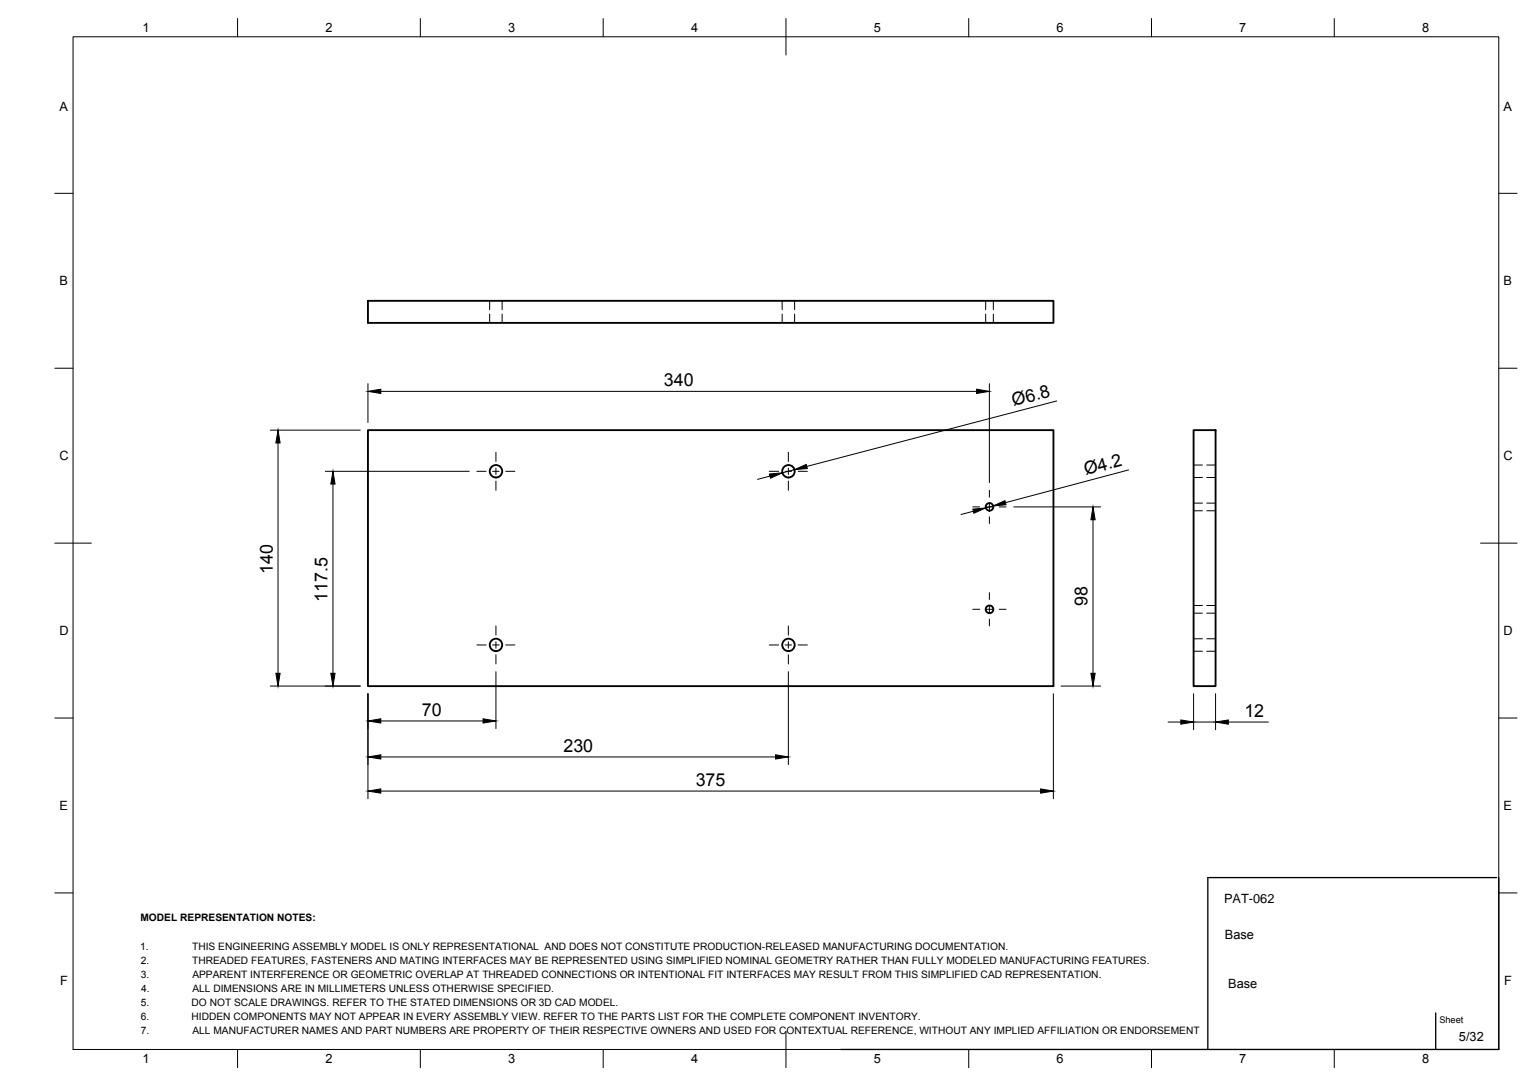
ISO-10303-21;
HEADER;
/* Generated by software containing ST-Developer
 * from STEP Tools, Inc. (www.steptools.com) 
 */

FILE_DESCRIPTION(
/* description */ ('Jaw-coupled motor to shaft test stand'),
/* implementation_level */ '2;1');

FILE_NAME(
/* name */ 'Base.step',
/* time_stamp */ '2026-10-27T10:46:06-07:00',
/* author */ (''),
/* organization */ (''),
/* preprocessor_version */ 'ST-DEVELOPER v20.2',
/* originating_system */ 'Autodesk Translation Framework v15.17.0.0',
/* authorisation */ '');

FILE_SCHEMA (('AUTOMOTIVE_DESIGN { 1 0 10303 214 3 1 1 }'));
ENDSEC;

DATA;
#10=MECHANICAL_DESIGN_GEOMETRIC_PRESENTATION_REPRESENTATION('',(#340),#19361);
#276=SHAPE_REPRESENTATION_RELATIONSHIP('SRR','None',#19490,#308);
#308=ADVANCED_BREP_SHAPE_REPRESENTATION('',(#373),#19326);
#340=STYLED_ITEM('',(#19725),#373);
#373=MANIFOLD_SOLID_BREP('Body1',#10984);
#403=FACE_BOUND('',#1653,.T.);
#404=FACE_BOUND('',#1654,.T.);
#405=FACE_BOUND('',#1655,.T.);
#406=FACE_BOUND('',#1656,.T.);
#407=FACE_BOUND('',#1657,.T.);
#408=FACE_BOUND('',#1658,.T.);
#409=FACE_BOUND('',#1660,.T.);
#410=FACE_BOUND('',#1661,.T.);
#411=FACE_BOUND('',#1662,.T.);
#412=FACE_BOUND('',#1663,.T.);
#413=FACE_BOUND('',#1664,.T.);
#414=FACE_BOUND('',#1665,.T.);
#516=PLANE('',#11394);
#517=PLANE('',#11395);
#518=PLANE('',#11396);
#519=PLANE('',#11397);
#520=PLANE('',#11398);
#521=PLANE('',#11399);
#1022=FACE_OUTER_BOUND('',#1642,.T.);
#1023=FACE_OUTER_BOUND('',#1643,.T.);
#1024=FACE_OUTER_BOUND('',#1644,.T.);
#1025=FACE_OUTER_BOUND('',#1645,.T.);
#1026=FACE_OUTER_BOUND('',#1646,.T.);
#1027=FACE_OUTER_BOUND('',#1647,.T.);
#1028=FACE_OUTER_BOUND('',#1648,.T.);
#1029=FACE_OUTER_BOUND('',#1649,.T.);
#1030=FACE_OUTER_BOUND('',#1650,.T.);
#1031=FACE_OUTER_BOUND('',#1651,.T.);
#1032=FACE_OUTER_BOUND('',#1652,.T.);
#1033=FACE_OUTER_BOUND('',#1659,.T.);
#1642=EDGE_LOOP('',(#7346,#7347,#7348,#7349));
#1643=EDGE_LOOP('',(#7350,#7351,#7352,#7353));
#1644=EDGE_LOOP('',(#7354,#7355,#7356,#7357));
#1645=EDGE_LOOP('',(#7358,#7359,#7360,#7361));
#1646=EDGE_LOOP('',(#7362,#7363,#7364,#7365));
#1647=EDGE_LOOP('',(#7366,#7367,#7368,#7369));
#1648=EDGE_LOOP('',(#7370,#7371,#7372,#7373));
#1649=EDGE_LOOP('',(#7374,#7375,#7376,#7377));
#1650=EDGE_LOOP('',(#7378,#7379,#7380,#7381));
#1651=EDGE_LOOP('',(#7382,#7383,#7384,#7385));
#1652=EDGE_LOOP('',(#7386,#7387,#7388,#7389));
#1653=EDGE_LOOP('',(#7390));
#1654=EDGE_LOOP('',(#7391));
#1655=EDGE_LOOP('',(#7392));
#1656=EDGE_LOOP('',(#7393));
#1657=EDGE_LOOP('',(#7394));
#1658=EDGE_LOOP('',(#7395));
#1659=EDGE_LOOP('',(#7396,#7397,#7398,#7399));
#1660=EDGE_LOOP('',(#7400));
#1661=EDGE_LOOP('',(#7401));
#1662=EDGE_LOOP('',(#7402));
#1663=EDGE_LOOP('',(#7403));
#1664=EDGE_LOOP('',(#7404));
#1665=EDGE_LOOP('',(#7405));
#2375=LINE('',#15434,#3528);
#2376=LINE('',#15440,#3529);
#2377=LINE('',#15446,#3530);
#2378=LINE('',#15452,#3531);
#2379=LINE('',#15458,#3532);
#2380=LINE('',#15464,#3533);
#2381=LINE('',#15469,#3534);
#2382=LINE('',#15471,#3535);
#2383=LINE('',#15473,#3536);
#2384=LINE('',#15474,#3537);
#2385=LINE('',#15477,#3538);
#2386=LINE('',#15479,#3539);
#2387=LINE('',#15480,#3540);
#2388=LINE('',#15483,#3541);
#2389=LINE('',#15485,#3542);
#2390=LINE('',#15486,#3543);
#2391=LINE('',#15488,#3544);
#2392=LINE('',#15489,#3545);
#3528=VECTOR('',#12350,0.21);
#3529=VECTOR('',#12357,0.21);
#3530=VECTOR('',#12364,0.34);
#3531=VECTOR('',#12371,0.34);
#3532=VECTOR('',#12378,0.34);
#3533=VECTOR('',#12385,0.34);
#3534=VECTOR('',#12390,1.);
#3535=VECTOR('',#12391,1.);
#3536=VECTOR('',#12392,1.);
#3537=VECTOR('',#12393,1.);
#3538=VECTOR('',#12396,1.);
#3539=VECTOR('',#12397,1.);
#3540=VECTOR('',#12398,1.);
#3541=VECTOR('',#12401,1.);
#3542=VECTOR('',#12402,1.);
#3543=VECTOR('',#12403,1.);
#3544=VECTOR('',#12406,1.);
#3545=VECTOR('',#12407,1.);
#4681=CIRCLE('',#11377,0.21);
#4682=CIRCLE('',#11378,0.21);
#4683=CIRCLE('',#11380,0.21);
#4684=CIRCLE('',#11381,0.21);
#4685=CIRCLE('',#11383,0.34);
#4686=CIRCLE('',#11384,0.34);
#4687=CIRCLE('',#11386,0.34);
#4688=CIRCLE('',#11387,0.34);
#4689=CIRCLE('',#11389,0.34);
#4690=CIRCLE('',#11390,0.34);
#4691=CIRCLE('',#11392,0.34);
#4692=CIRCLE('',#11393,0.34);
#4943=VERTEX_POINT('',#15431);
#4944=VERTEX_POINT('',#15433);
#4945=VERTEX_POINT('',#15437);
#4946=VERTEX_POINT('',#15439);
#4947=VERTEX_POINT('',#15443);
#4948=VERTEX_POINT('',#15445);
#4949=VERTEX_POINT('',#15449);
#4950=VERTEX_POINT('',#15451);
#4951=VERTEX_POINT('',#15455);
#4952=VERTEX_POINT('',#15457);
#4953=VERTEX_POINT('',#15461);
#4954=VERTEX_POINT('',#15463);
#4955=VERTEX_POINT('',#15467);
#4956=VERTEX_POINT('',#15468);
#4957=VERTEX_POINT('',#15470);
#4958=VERTEX_POINT('',#15472);
#4959=VERTEX_POINT('',#15476);
#4960=VERTEX_POINT('',#15478);
#4961=VERTEX_POINT('',#15482);
#4962=VERTEX_POINT('',#15484);
#5884=EDGE_CURVE('',#4943,#4943,#4681,.T.);
#5885=EDGE_CURVE('',#4943,#4944,#2375,.T.);
#5886=EDGE_CURVE('',#4944,#4944,#4682,.T.);
#5887=EDGE_CURVE('',#4945,#4945,#4683,.T.);
#5888=EDGE_CURVE('',#4945,#4946,#2376,.T.);
#5889=EDGE_CURVE('',#4946,#4946,#4684,.T.);
#5890=EDGE_CURVE('',#4947,#4947,#4685,.T.);
#5891=EDGE_CURVE('',#4947,#4948,#2377,.T.);
#5892=EDGE_CURVE('',#4948,#4948,#4686,.T.);
#5893=EDGE_CURVE('',#4949,#4949,#4687,.T.);
#5894=EDGE_CURVE('',#4949,#4950,#2378,.T.);
#5895=EDGE_CURVE('',#4950,#4950,#4688,.T.);
#5896=EDGE_CURVE('',#4951,#4951,#4689,.T.);
#5897=EDGE_CURVE('',#4951,#4952,#2379,.T.);
#5898=EDGE_CURVE('',#4952,#4952,#4690,.T.);
#5899=EDGE_CURVE('',#4953,#4953,#4691,.T.);
#5900=EDGE_CURVE('',#4953,#4954,#2380,.T.);
#5901=EDGE_CURVE('',#4954,#4954,#4692,.T.);
#5902=EDGE_CURVE('',#4955,#4956,#2381,.T.);
#5903=EDGE_CURVE('',#4956,#4957,#2382,.T.);
#5904=EDGE_CURVE('',#4958,#4957,#2383,.T.);
#5905=EDGE_CURVE('',#4955,#4958,#2384,.T.);
#5906=EDGE_CURVE('',#4959,#4955,#2385,.T.);
#5907=EDGE_CURVE('',#4960,#4958,#2386,.T.);
#5908=EDGE_CURVE('',#4959,#4960,#2387,.T.);
#5909=EDGE_CURVE('',#4961,#4959,#2388,.T.);
#5910=EDGE_CURVE('',#4962,#4960,#2389,.T.);
#5911=EDGE_CURVE('',#4961,#4962,#2390,.T.);
#5912=EDGE_CURVE('',#4956,#4961,#2391,.T.);
#5913=EDGE_CURVE('',#4957,#4962,#2392,.T.);
#7346=ORIENTED_EDGE('',*,*,#5884,.F.);
#7347=ORIENTED_EDGE('',*,*,#5885,.T.);
#7348=ORIENTED_EDGE('',*,*,#5886,.F.);
#7349=ORIENTED_EDGE('',*,*,#5885,.F.);
#7350=ORIENTED_EDGE('',*,*,#5887,.F.);
#7351=ORIENTED_EDGE('',*,*,#5888,.T.);
#7352=ORIENTED_EDGE('',*,*,#5889,.F.);
#7353=ORIENTED_EDGE('',*,*,#5888,.F.);
#7354=ORIENTED_EDGE('',*,*,#5890,.F.);
#7355=ORIENTED_EDGE('',*,*,#5891,.T.);
#7356=ORIENTED_EDGE('',*,*,#5892,.F.);
#7357=ORIENTED_EDGE('',*,*,#5891,.F.);
#7358=ORIENTED_EDGE('',*,*,#5893,.F.);
#7359=ORIENTED_EDGE('',*,*,#5894,.T.);
#7360=ORIENTED_EDGE('',*,*,#5895,.F.);
#7361=ORIENTED_EDGE('',*,*,#5894,.F.);
#7362=ORIENTED_EDGE('',*,*,#5896,.F.);
#7363=ORIENTED_EDGE('',*,*,#5897,.T.);
#7364=ORIENTED_EDGE('',*,*,#5898,.F.);
#7365=ORIENTED_EDGE('',*,*,#5897,.F.);
#7366=ORIENTED_EDGE('',*,*,#5899,.F.);
#7367=ORIENTED_EDGE('',*,*,#5900,.T.);
#7368=ORIENTED_EDGE('',*,*,#5901,.F.);
#7369=ORIENTED_EDGE('',*,*,#5900,.F.);
#7370=ORIENTED_EDGE('',*,*,#5902,.T.);
#7371=ORIENTED_EDGE('',*,*,#5903,.T.);
#7372=ORIENTED_EDGE('',*,*,#5904,.F.);
#7373=ORIENTED_EDGE('',*,*,#5905,.F.);
#7374=ORIENTED_EDGE('',*,*,#5906,.T.);
#7375=ORIENTED_EDGE('',*,*,#5905,.T.);
#7376=ORIENTED_EDGE('',*,*,#5907,.F.);
#7377=ORIENTED_EDGE('',*,*,#5908,.F.);
#7378=ORIENTED_EDGE('',*,*,#5909,.T.);
#7379=ORIENTED_EDGE('',*,*,#5908,.T.);
#7380=ORIENTED_EDGE('',*,*,#5910,.F.);
#7381=ORIENTED_EDGE('',*,*,#5911,.F.);
#7382=ORIENTED_EDGE('',*,*,#5912,.T.);
#7383=ORIENTED_EDGE('',*,*,#5911,.T.);
#7384=ORIENTED_EDGE('',*,*,#5913,.F.);
#7385=ORIENTED_EDGE('',*,*,#5903,.F.);
#7386=ORIENTED_EDGE('',*,*,#5913,.T.);
#7387=ORIENTED_EDGE('',*,*,#5910,.T.);
#7388=ORIENTED_EDGE('',*,*,#5907,.T.);
#7389=ORIENTED_EDGE('',*,*,#5904,.T.);
#7390=ORIENTED_EDGE('',*,*,#5886,.T.);
#7391=ORIENTED_EDGE('',*,*,#5889,.T.);
#7392=ORIENTED_EDGE('',*,*,#5892,.T.);
#7393=ORIENTED_EDGE('',*,*,#5895,.T.);
#7394=ORIENTED_EDGE('',*,*,#5898,.T.);
#7395=ORIENTED_EDGE('',*,*,#5901,.T.);
#7396=ORIENTED_EDGE('',*,*,#5912,.F.);
#7397=ORIENTED_EDGE('',*,*,#5902,.F.);
#7398=ORIENTED_EDGE('',*,*,#5906,.F.);
#7399=ORIENTED_EDGE('',*,*,#5909,.F.);
#7400=ORIENTED_EDGE('',*,*,#5884,.T.);
#7401=ORIENTED_EDGE('',*,*,#5887,.T.);
#7402=ORIENTED_EDGE('',*,*,#5890,.T.);
#7403=ORIENTED_EDGE('',*,*,#5893,.T.);
#7404=ORIENTED_EDGE('',*,*,#5896,.T.);
#7405=ORIENTED_EDGE('',*,*,#5899,.T.);
#10270=CYLINDRICAL_SURFACE('',#11376,0.21);
#10271=CYLINDRICAL_SURFACE('',#11379,0.21);
#10272=CYLINDRICAL_SURFACE('',#11382,0.34);
#10273=CYLINDRICAL_SURFACE('',#11385,0.34);
#10274=CYLINDRICAL_SURFACE('',#11388,0.34);
#10275=CYLINDRICAL_SURFACE('',#11391,0.34);
#10364=ADVANCED_FACE('',(#1022),#10270,.F.);
#10365=ADVANCED_FACE('',(#1023),#10271,.F.);
#10366=ADVANCED_FACE('',(#1024),#10272,.F.);
#10367=ADVANCED_FACE('',(#1025),#10273,.F.);
#10368=ADVANCED_FACE('',(#1026),#10274,.F.);
#10369=ADVANCED_FACE('',(#1027),#10275,.F.);
#10370=ADVANCED_FACE('',(#1028),#516,.T.);
#10371=ADVANCED_FACE('',(#1029),#517,.T.);
#10372=ADVANCED_FACE('',(#1030),#518,.T.);
#10373=ADVANCED_FACE('',(#1031),#519,.T.);
#10374=ADVANCED_FACE('',(#1032,#403,#404,#405,#406,#407,#408),#520,.T.);
#10375=ADVANCED_FACE('',(#1033,#409,#410,#411,#412,#413,#414),#521,.F.);
#10984=CLOSED_SHELL('',(#10364,#10365,#10366,#10367,#10368,#10369,#10370,
#10371,#10372,#10373,#10374,#10375));
#11375=AXIS2_PLACEMENT_3D('',#15429,#12344,#12345);
#11376=AXIS2_PLACEMENT_3D('',#15430,#12346,#12347);
#11377=AXIS2_PLACEMENT_3D('',#15432,#12348,#12349);
#11378=AXIS2_PLACEMENT_3D('',#15435,#12351,#12352);
#11379=AXIS2_PLACEMENT_3D('',#15436,#12353,#12354);
#11380=AXIS2_PLACEMENT_3D('',#15438,#12355,#12356);
#11381=AXIS2_PLACEMENT_3D('',#15441,#12358,#12359);
#11382=AXIS2_PLACEMENT_3D('',#15442,#12360,#12361);
#11383=AXIS2_PLACEMENT_3D('',#15444,#12362,#12363);
#11384=AXIS2_PLACEMENT_3D('',#15447,#12365,#12366);
#11385=AXIS2_PLACEMENT_3D('',#15448,#12367,#12368);
#11386=AXIS2_PLACEMENT_3D('',#15450,#12369,#12370);
#11387=AXIS2_PLACEMENT_3D('',#15453,#12372,#12373);
#11388=AXIS2_PLACEMENT_3D('',#15454,#12374,#12375);
#11389=AXIS2_PLACEMENT_3D('',#15456,#12376,#12377);
#11390=AXIS2_PLACEMENT_3D('',#15459,#12379,#12380);
#11391=AXIS2_PLACEMENT_3D('',#15460,#12381,#12382);
#11392=AXIS2_PLACEMENT_3D('',#15462,#12383,#12384);
#11393=AXIS2_PLACEMENT_3D('',#15465,#12386,#12387);
#11394=AXIS2_PLACEMENT_3D('',#15466,#12388,#12389);
#11395=AXIS2_PLACEMENT_3D('',#15475,#12394,#12395);
#11396=AXIS2_PLACEMENT_3D('',#15481,#12399,#12400);
#11397=AXIS2_PLACEMENT_3D('',#15487,#12404,#12405);
#11398=AXIS2_PLACEMENT_3D('',#15490,#12408,#12409);
#11399=AXIS2_PLACEMENT_3D('',#15491,#12410,#12411);
#12344=DIRECTION('axis',(0.,0.,1.));
#12345=DIRECTION('refdir',(1.,0.,0.));
#12346=DIRECTION('center_axis',(0.,0.,1.));
#12347=DIRECTION('ref_axis',(1.,0.,0.));
#12348=DIRECTION('center_axis',(0.,0.,1.));
#12349=DIRECTION('ref_axis',(1.,0.,0.));
#12350=DIRECTION('',(0.,0.,1.));
#12351=DIRECTION('center_axis',(0.,0.,-1.));
#12352=DIRECTION('ref_axis',(1.,0.,0.));
#12353=DIRECTION('center_axis',(0.,0.,1.));
#12354=DIRECTION('ref_axis',(1.,0.,0.));
#12355=DIRECTION('center_axis',(0.,0.,1.));
#12356=DIRECTION('ref_axis',(1.,0.,0.));
#12357=DIRECTION('',(0.,0.,1.));
#12358=DIRECTION('center_axis',(0.,0.,-1.));
#12359=DIRECTION('ref_axis',(1.,0.,0.));
#12360=DIRECTION('center_axis',(0.,0.,1.));
#12361=DIRECTION('ref_axis',(1.,0.,0.));
#12362=DIRECTION('center_axis',(0.,0.,1.));
#12363=DIRECTION('ref_axis',(1.,0.,0.));
#12364=DIRECTION('',(0.,0.,1.));
#12365=DIRECTION('center_axis',(0.,0.,-1.));
#12366=DIRECTION('ref_axis',(1.,0.,0.));
#12367=DIRECTION('center_axis',(0.,0.,1.));
#12368=DIRECTION('ref_axis',(1.,0.,0.));
#12369=DIRECTION('center_axis',(0.,0.,1.));
#12370=DIRECTION('ref_axis',(1.,0.,0.));
#12371=DIRECTION('',(0.,0.,1.));
#12372=DIRECTION('center_axis',(0.,0.,-1.));
#12373=DIRECTION('ref_axis',(1.,0.,0.));
#12374=DIRECTION('center_axis',(0.,0.,1.));
#12375=DIRECTION('ref_axis',(1.,0.,0.));
#12376=DIRECTION('center_axis',(0.,0.,1.));
#12377=DIRECTION('ref_axis',(1.,0.,0.));
#12378=DIRECTION('',(0.,0.,1.));
#12379=DIRECTION('center_axis',(0.,0.,-1.));
#12380=DIRECTION('ref_axis',(1.,0.,0.));
#12381=DIRECTION('center_axis',(0.,0.,1.));
#12382=DIRECTION('ref_axis',(1.,0.,0.));
#12383=DIRECTION('center_axis',(0.,0.,1.));
#12384=DIRECTION('ref_axis',(1.,0.,0.));
#12385=DIRECTION('',(0.,0.,1.));
#12386=DIRECTION('center_axis',(0.,0.,-1.));
#12387=DIRECTION('ref_axis',(1.,0.,0.));
#12388=DIRECTION('center_axis',(0.,1.,0.));
#12389=DIRECTION('ref_axis',(-1.,0.,0.));
#12390=DIRECTION('',(-1.,0.,0.));
#12391=DIRECTION('',(0.,0.,1.));
#12392=DIRECTION('',(-1.,0.,0.));
#12393=DIRECTION('',(0.,0.,1.));
#12394=DIRECTION('center_axis',(1.,0.,0.));
#12395=DIRECTION('ref_axis',(0.,1.,0.));
#12396=DIRECTION('',(0.,1.,0.));
#12397=DIRECTION('',(0.,1.,0.));
#12398=DIRECTION('',(0.,0.,1.));
#12399=DIRECTION('center_axis',(0.,-1.,0.));
#12400=DIRECTION('ref_axis',(1.,0.,0.));
#12401=DIRECTION('',(1.,0.,0.));
#12402=DIRECTION('',(1.,0.,0.));
#12403=DIRECTION('',(0.,0.,1.));
#12404=DIRECTION('center_axis',(-1.,0.,0.));
#12405=DIRECTION('ref_axis',(0.,-1.,0.));
#12406=DIRECTION('',(0.,-1.,0.));
#12407=DIRECTION('',(0.,-1.,0.));
#12408=DIRECTION('center_axis',(0.,0.,1.));
#12409=DIRECTION('ref_axis',(1.,0.,0.));
#12410=DIRECTION('center_axis',(0.,0.,1.));
#12411=DIRECTION('ref_axis',(1.,0.,0.));
#15429=CARTESIAN_POINT('',(0.,0.,0.));
#15430=CARTESIAN_POINT('Origin',(-2.8,-9.,-0.1));
#15431=CARTESIAN_POINT('',(-3.01,-9.,0.));
#15432=CARTESIAN_POINT('Origin',(-2.8,-9.,0.));
#15433=CARTESIAN_POINT('',(-3.01,-9.,1.2));
#15434=CARTESIAN_POINT('',(-3.01,-9.,-0.1));
#15435=CARTESIAN_POINT('Origin',(-2.8,-9.,1.2));
#15436=CARTESIAN_POINT('Origin',(2.8,-9.,-0.1));
#15437=CARTESIAN_POINT('',(2.59,-9.,0.));
#15438=CARTESIAN_POINT('Origin',(2.8,-9.,0.));
#15439=CARTESIAN_POINT('',(2.59,-9.,1.2));
#15440=CARTESIAN_POINT('',(2.59,-9.,-0.1));
#15441=CARTESIAN_POINT('Origin',(2.8,-9.,1.2));
#15442=CARTESIAN_POINT('Origin',(4.75,2.,-0.1));
#15443=CARTESIAN_POINT('',(4.41,2.,0.));
#15444=CARTESIAN_POINT('Origin',(4.75,2.,0.));
#15445=CARTESIAN_POINT('',(4.41,2.,1.2));
#15446=CARTESIAN_POINT('',(4.41,2.,-0.1));
#15447=CARTESIAN_POINT('Origin',(4.75,2.,1.2));
#15448=CARTESIAN_POINT('Origin',(-4.75,18.,-0.1));
#15449=CARTESIAN_POINT('',(-5.09,18.,0.));
#15450=CARTESIAN_POINT('Origin',(-4.75,18.,0.));
#15451=CARTESIAN_POINT('',(-5.09,18.,1.2));
#15452=CARTESIAN_POINT('',(-5.09,18.,-0.1));
#15453=CARTESIAN_POINT('Origin',(-4.75,18.,1.2));
#15454=CARTESIAN_POINT('Origin',(-4.75,2.,-0.1));
#15455=CARTESIAN_POINT('',(-5.09,2.,0.));
#15456=CARTESIAN_POINT('Origin',(-4.75,2.,0.));
#15457=CARTESIAN_POINT('',(-5.09,2.,1.2));
#15458=CARTESIAN_POINT('',(-5.09,2.,-0.1));
#15459=CARTESIAN_POINT('Origin',(-4.75,2.,1.2));
#15460=CARTESIAN_POINT('Origin',(4.75,18.,-0.1));
#15461=CARTESIAN_POINT('',(4.41,18.,0.));
#15462=CARTESIAN_POINT('Origin',(4.75,18.,0.));
#15463=CARTESIAN_POINT('',(4.41,18.,1.2));
#15464=CARTESIAN_POINT('',(4.41,18.,-0.1));
#15465=CARTESIAN_POINT('Origin',(4.75,18.,1.2));
#15466=CARTESIAN_POINT('Origin',(7.,25.,0.));
#15467=CARTESIAN_POINT('',(7.,25.,0.));
#15468=CARTESIAN_POINT('',(-7.,25.,0.));
#15469=CARTESIAN_POINT('',(7.,25.,0.));
#15470=CARTESIAN_POINT('',(-7.,25.,1.2));
#15471=CARTESIAN_POINT('',(-7.,25.,0.));
#15472=CARTESIAN_POINT('',(7.,25.,1.2));
#15473=CARTESIAN_POINT('',(7.,25.,1.2));
#15474=CARTESIAN_POINT('',(7.,25.,0.));
#15475=CARTESIAN_POINT('Origin',(7.,-12.5,0.));
#15476=CARTESIAN_POINT('',(7.,-12.5,0.));
#15477=CARTESIAN_POINT('',(7.,-12.5,0.));
#15478=CARTESIAN_POINT('',(7.,-12.5,1.2));
#15479=CARTESIAN_POINT('',(7.,-12.5,1.2));
#15480=CARTESIAN_POINT('',(7.,-12.5,0.));
#15481=CARTESIAN_POINT('Origin',(-7.,-12.5,0.));
#15482=CARTESIAN_POINT('',(-7.,-12.5,0.));
#15483=CARTESIAN_POINT('',(-7.,-12.5,0.));
#15484=CARTESIAN_POINT('',(-7.,-12.5,1.2));
#15485=CARTESIAN_POINT('',(-7.,-12.5,1.2));
#15486=CARTESIAN_POINT('',(-7.,-12.5,0.));
#15487=CARTESIAN_POINT('Origin',(-7.,25.,0.));
#15488=CARTESIAN_POINT('',(-7.,25.,0.));
#15489=CARTESIAN_POINT('',(-7.,25.,1.2));
#15490=CARTESIAN_POINT('Origin',(0.,6.25,1.2));
#15491=CARTESIAN_POINT('Origin',(0.,6.25,0.));
#19288=UNCERTAINTY_MEASURE_WITH_UNIT(LENGTH_MEASURE(0.001),#19362,
'DISTANCE_ACCURACY_VALUE',
'Maximum model space distance between geometric entities at asserted c
onnectivities');
#19323=UNCERTAINTY_MEASURE_WITH_UNIT(LENGTH_MEASURE(0.001),#19362,
'DISTANCE_ACCURACY_VALUE',
'Maximum model space distance between geometric entities at asserted c
onnectivities');
#19326=(
GEOMETRIC_REPRESENTATION_CONTEXT(3)
GLOBAL_UNCERTAINTY_ASSIGNED_CONTEXT((#19288))
GLOBAL_UNIT_ASSIGNED_CONTEXT((#19362,#19364,#19365))
REPRESENTATION_CONTEXT('','3D')
);
#19361=(
GEOMETRIC_REPRESENTATION_CONTEXT(3)
GLOBAL_UNCERTAINTY_ASSIGNED_CONTEXT((#19323))
GLOBAL_UNIT_ASSIGNED_CONTEXT((#19362,#19364,#19365))
REPRESENTATION_CONTEXT('','3D')
);
#19362=(
LENGTH_UNIT()
NAMED_UNIT(*)
SI_UNIT(.CENTI.,.METRE.)
);
#19364=(
NAMED_UNIT(*)
PLANE_ANGLE_UNIT()
SI_UNIT($,.RADIAN.)
);
#19365=(
NAMED_UNIT(*)
SI_UNIT($,.STERADIAN.)
SOLID_ANGLE_UNIT()
);
#19368=SHAPE_DEFINITION_REPRESENTATION(#19405,#19490);
#19405=PRODUCT_DEFINITION_SHAPE('',$,#19528);
#19490=SHAPE_REPRESENTATION('',(#11375),#19326);
#19525=PRODUCT_DEFINITION_CONTEXT('part definition',#19638,'design');
#19528=PRODUCT_DEFINITION('Base','Base',#19565,#19525);
#19565=PRODUCT_DEFINITION_FORMATION('',$,#19642);
#19638=APPLICATION_CONTEXT(
'Core Data for Automotive Mechanical Design Process');
#19639=PRODUCT_CONTEXT('part definition',#19638,'mechanical');
#19642=PRODUCT('Base','Base','Base',(#19639));
#19719=COLOUR_RGB('Dark Blue',0.08,0.2,0.34);
#19720=FILL_AREA_STYLE_COLOUR('',#19719);
#19721=FILL_AREA_STYLE('',(#19720));
#19722=SURFACE_STYLE_FILL_AREA(#19721);
#19723=SURFACE_SIDE_STYLE('',(#19722));
#19724=SURFACE_STYLE_USAGE(.BOTH.,#19723);
#19725=PRESENTATION_STYLE_ASSIGNMENT((#19724));
ENDSEC;
END-ISO-10303-21;
